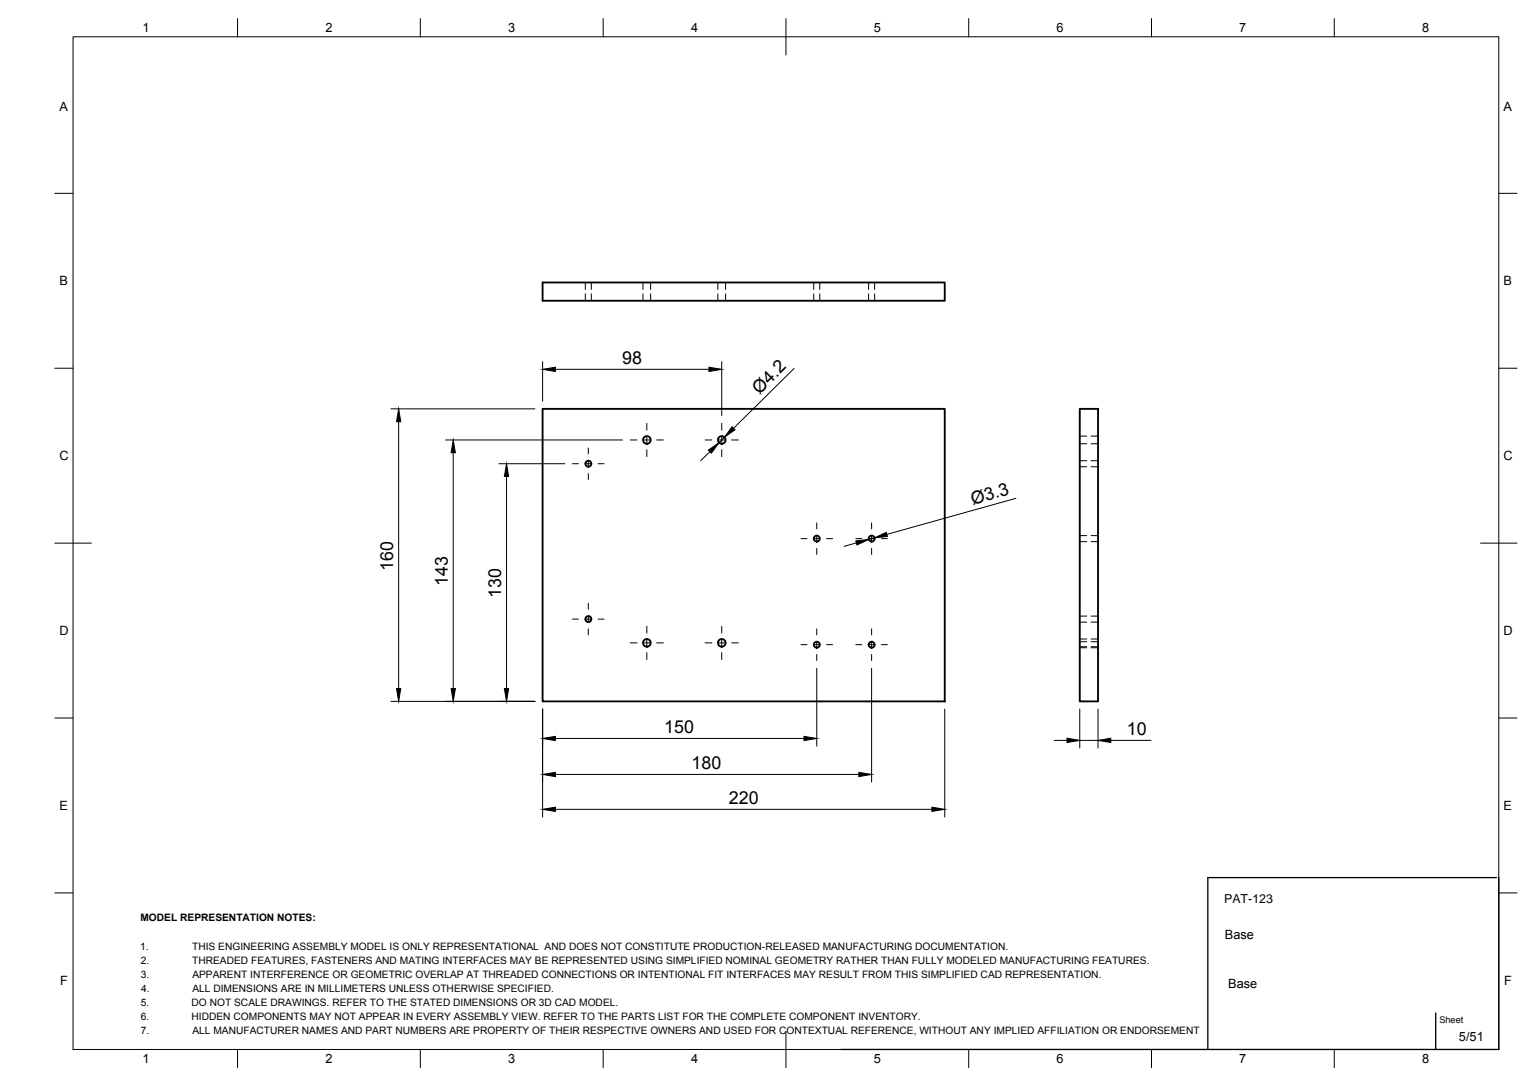
ISO-10303-21;
HEADER;
/* Generated by software containing ST-Developer
 * from STEP Tools, Inc. (www.steptools.com) 
 */

FILE_DESCRIPTION(
/* description */ ('Worm-less right-angle friction wheel drive'),
/* implementation_level */ '2;1');

FILE_NAME(
/* name */ 'Base.step',
/* time_stamp */ '2026-10-28T03:22:36-07:00',
/* author */ (''),
/* organization */ (''),
/* preprocessor_version */ 'ST-DEVELOPER v20.2',
/* originating_system */ 'Autodesk Translation Framework v15.17.0.0',
/* authorisation */ '');

FILE_SCHEMA (('AUTOMOTIVE_DESIGN { 1 0 10303 214 3 1 1 }'));
ENDSEC;

DATA;
#10=MECHANICAL_DESIGN_GEOMETRIC_PRESENTATION_REPRESENTATION('',(#611),#17046);
#517=SHAPE_REPRESENTATION_RELATIONSHIP('SRR','None',#17260,#564);
#564=ADVANCED_BREP_SHAPE_REPRESENTATION('',(#665),#16996);
#611=STYLED_ITEM('',(#17570),#665);
#665=MANIFOLD_SOLID_BREP('Body1',#8166);
#715=FACE_BOUND('',#1689,.T.);
#716=FACE_BOUND('',#1690,.T.);
#717=FACE_BOUND('',#1691,.T.);
#718=FACE_BOUND('',#1692,.T.);
#719=FACE_BOUND('',#1693,.T.);
#720=FACE_BOUND('',#1694,.T.);
#721=FACE_BOUND('',#1695,.T.);
#722=FACE_BOUND('',#1696,.T.);
#723=FACE_BOUND('',#1697,.T.);
#724=FACE_BOUND('',#1698,.T.);
#725=FACE_BOUND('',#1700,.T.);
#726=FACE_BOUND('',#1701,.T.);
#727=FACE_BOUND('',#1702,.T.);
#728=FACE_BOUND('',#1703,.T.);
#729=FACE_BOUND('',#1704,.T.);
#730=FACE_BOUND('',#1705,.T.);
#731=FACE_BOUND('',#1706,.T.);
#732=FACE_BOUND('',#1707,.T.);
#733=FACE_BOUND('',#1708,.T.);
#734=FACE_BOUND('',#1709,.T.);
#952=PLANE('',#8775);
#953=PLANE('',#8776);
#954=PLANE('',#8777);
#955=PLANE('',#8778);
#956=PLANE('',#8779);
#957=PLANE('',#8780);
#1208=FACE_OUTER_BOUND('',#1674,.T.);
#1209=FACE_OUTER_BOUND('',#1675,.T.);
#1210=FACE_OUTER_BOUND('',#1676,.T.);
#1211=FACE_OUTER_BOUND('',#1677,.T.);
#1212=FACE_OUTER_BOUND('',#1678,.T.);
#1213=FACE_OUTER_BOUND('',#1679,.T.);
#1214=FACE_OUTER_BOUND('',#1680,.T.);
#1215=FACE_OUTER_BOUND('',#1681,.T.);
#1216=FACE_OUTER_BOUND('',#1682,.T.);
#1217=FACE_OUTER_BOUND('',#1683,.T.);
#1218=FACE_OUTER_BOUND('',#1684,.T.);
#1219=FACE_OUTER_BOUND('',#1685,.T.);
#1220=FACE_OUTER_BOUND('',#1686,.T.);
#1221=FACE_OUTER_BOUND('',#1687,.T.);
#1222=FACE_OUTER_BOUND('',#1688,.T.);
#1223=FACE_OUTER_BOUND('',#1699,.T.);
#1674=EDGE_LOOP('',(#5534,#5535,#5536,#5537));
#1675=EDGE_LOOP('',(#5538,#5539,#5540,#5541));
#1676=EDGE_LOOP('',(#5542,#5543,#5544,#5545));
#1677=EDGE_LOOP('',(#5546,#5547,#5548,#5549));
#1678=EDGE_LOOP('',(#5550,#5551,#5552,#5553));
#1679=EDGE_LOOP('',(#5554,#5555,#5556,#5557));
#1680=EDGE_LOOP('',(#5558,#5559,#5560,#5561));
#1681=EDGE_LOOP('',(#5562,#5563,#5564,#5565));
#1682=EDGE_LOOP('',(#5566,#5567,#5568,#5569));
#1683=EDGE_LOOP('',(#5570,#5571,#5572,#5573));
#1684=EDGE_LOOP('',(#5574,#5575,#5576,#5577));
#1685=EDGE_LOOP('',(#5578,#5579,#5580,#5581));
#1686=EDGE_LOOP('',(#5582,#5583,#5584,#5585));
#1687=EDGE_LOOP('',(#5586,#5587,#5588,#5589));
#1688=EDGE_LOOP('',(#5590,#5591,#5592,#5593));
#1689=EDGE_LOOP('',(#5594));
#1690=EDGE_LOOP('',(#5595));
#1691=EDGE_LOOP('',(#5596));
#1692=EDGE_LOOP('',(#5597));
#1693=EDGE_LOOP('',(#5598));
#1694=EDGE_LOOP('',(#5599));
#1695=EDGE_LOOP('',(#5600));
#1696=EDGE_LOOP('',(#5601));
#1697=EDGE_LOOP('',(#5602));
#1698=EDGE_LOOP('',(#5603));
#1699=EDGE_LOOP('',(#5604,#5605,#5606,#5607));
#1700=EDGE_LOOP('',(#5608));
#1701=EDGE_LOOP('',(#5609));
#1702=EDGE_LOOP('',(#5610));
#1703=EDGE_LOOP('',(#5611));
#1704=EDGE_LOOP('',(#5612));
#1705=EDGE_LOOP('',(#5613));
#1706=EDGE_LOOP('',(#5614));
#1707=EDGE_LOOP('',(#5615));
#1708=EDGE_LOOP('',(#5616));
#1709=EDGE_LOOP('',(#5617));
#2377=LINE('',#12382,#2917);
#2378=LINE('',#12388,#2918);
#2379=LINE('',#12394,#2919);
#2380=LINE('',#12400,#2920);
#2381=LINE('',#12406,#2921);
#2382=LINE('',#12412,#2922);
#2383=LINE('',#12418,#2923);
#2384=LINE('',#12424,#2924);
#2385=LINE('',#12430,#2925);
#2386=LINE('',#12436,#2926);
#2387=LINE('',#12441,#2927);
#2388=LINE('',#12443,#2928);
#2389=LINE('',#12445,#2929);
#2390=LINE('',#12446,#2930);
#2391=LINE('',#12449,#2931);
#2392=LINE('',#12451,#2932);
#2393=LINE('',#12452,#2933);
#2394=LINE('',#12455,#2934);
#2395=LINE('',#12457,#2935);
#2396=LINE('',#12458,#2936);
#2397=LINE('',#12460,#2937);
#2398=LINE('',#12461,#2938);
#2917=VECTOR('',#9783,0.165);
#2918=VECTOR('',#9790,0.165);
#2919=VECTOR('',#9797,0.165);
#2920=VECTOR('',#9804,0.165);
#2921=VECTOR('',#9811,0.165);
#2922=VECTOR('',#9818,0.165);
#2923=VECTOR('',#9825,0.210000000000001);
#2924=VECTOR('',#9832,0.21);
#2925=VECTOR('',#9839,0.21);
#2926=VECTOR('',#9846,0.210000000000001);
#2927=VECTOR('',#9851,1.);
#2928=VECTOR('',#9852,1.);
#2929=VECTOR('',#9853,1.);
#2930=VECTOR('',#9854,1.);
#2931=VECTOR('',#9857,1.);
#2932=VECTOR('',#9858,1.);
#2933=VECTOR('',#9859,1.);
#2934=VECTOR('',#9862,1.);
#2935=VECTOR('',#9863,1.);
#2936=VECTOR('',#9864,1.);
#2937=VECTOR('',#9867,1.);
#2938=VECTOR('',#9868,1.);
#3457=CIRCLE('',#8746,0.165);
#3458=CIRCLE('',#8747,0.165);
#3459=CIRCLE('',#8749,0.165);
#3460=CIRCLE('',#8750,0.165);
#3461=CIRCLE('',#8752,0.165);
#3462=CIRCLE('',#8753,0.165);
#3463=CIRCLE('',#8755,0.165);
#3464=CIRCLE('',#8756,0.165);
#3465=CIRCLE('',#8758,0.165);
#3466=CIRCLE('',#8759,0.165);
#3467=CIRCLE('',#8761,0.165);
#3468=CIRCLE('',#8762,0.165);
#3469=CIRCLE('',#8764,0.210000000000001);
#3470=CIRCLE('',#8765,0.210000000000001);
#3471=CIRCLE('',#8767,0.21);
#3472=CIRCLE('',#8768,0.21);
#3473=CIRCLE('',#8770,0.21);
#3474=CIRCLE('',#8771,0.21);
#3475=CIRCLE('',#8773,0.210000000000001);
#3476=CIRCLE('',#8774,0.210000000000001);
#3869=VERTEX_POINT('',#12379);
#3870=VERTEX_POINT('',#12381);
#3871=VERTEX_POINT('',#12385);
#3872=VERTEX_POINT('',#12387);
#3873=VERTEX_POINT('',#12391);
#3874=VERTEX_POINT('',#12393);
#3875=VERTEX_POINT('',#12397);
#3876=VERTEX_POINT('',#12399);
#3877=VERTEX_POINT('',#12403);
#3878=VERTEX_POINT('',#12405);
#3879=VERTEX_POINT('',#12409);
#3880=VERTEX_POINT('',#12411);
#3881=VERTEX_POINT('',#12415);
#3882=VERTEX_POINT('',#12417);
#3883=VERTEX_POINT('',#12421);
#3884=VERTEX_POINT('',#12423);
#3885=VERTEX_POINT('',#12427);
#3886=VERTEX_POINT('',#12429);
#3887=VERTEX_POINT('',#12433);
#3888=VERTEX_POINT('',#12435);
#3889=VERTEX_POINT('',#12439);
#3890=VERTEX_POINT('',#12440);
#3891=VERTEX_POINT('',#12442);
#3892=VERTEX_POINT('',#12444);
#3893=VERTEX_POINT('',#12448);
#3894=VERTEX_POINT('',#12450);
#3895=VERTEX_POINT('',#12454);
#3896=VERTEX_POINT('',#12456);
#4536=EDGE_CURVE('',#3869,#3869,#3457,.T.);
#4537=EDGE_CURVE('',#3869,#3870,#2377,.T.);
#4538=EDGE_CURVE('',#3870,#3870,#3458,.T.);
#4539=EDGE_CURVE('',#3871,#3871,#3459,.T.);
#4540=EDGE_CURVE('',#3871,#3872,#2378,.T.);
#4541=EDGE_CURVE('',#3872,#3872,#3460,.T.);
#4542=EDGE_CURVE('',#3873,#3873,#3461,.T.);
#4543=EDGE_CURVE('',#3873,#3874,#2379,.T.);
#4544=EDGE_CURVE('',#3874,#3874,#3462,.T.);
#4545=EDGE_CURVE('',#3875,#3875,#3463,.T.);
#4546=EDGE_CURVE('',#3875,#3876,#2380,.T.);
#4547=EDGE_CURVE('',#3876,#3876,#3464,.T.);
#4548=EDGE_CURVE('',#3877,#3877,#3465,.T.);
#4549=EDGE_CURVE('',#3877,#3878,#2381,.T.);
#4550=EDGE_CURVE('',#3878,#3878,#3466,.T.);
#4551=EDGE_CURVE('',#3879,#3879,#3467,.T.);
#4552=EDGE_CURVE('',#3879,#3880,#2382,.T.);
#4553=EDGE_CURVE('',#3880,#3880,#3468,.T.);
#4554=EDGE_CURVE('',#3881,#3881,#3469,.T.);
#4555=EDGE_CURVE('',#3881,#3882,#2383,.T.);
#4556=EDGE_CURVE('',#3882,#3882,#3470,.T.);
#4557=EDGE_CURVE('',#3883,#3883,#3471,.T.);
#4558=EDGE_CURVE('',#3883,#3884,#2384,.T.);
#4559=EDGE_CURVE('',#3884,#3884,#3472,.T.);
#4560=EDGE_CURVE('',#3885,#3885,#3473,.T.);
#4561=EDGE_CURVE('',#3885,#3886,#2385,.T.);
#4562=EDGE_CURVE('',#3886,#3886,#3474,.T.);
#4563=EDGE_CURVE('',#3887,#3887,#3475,.T.);
#4564=EDGE_CURVE('',#3887,#3888,#2386,.T.);
#4565=EDGE_CURVE('',#3888,#3888,#3476,.T.);
#4566=EDGE_CURVE('',#3889,#3890,#2387,.T.);
#4567=EDGE_CURVE('',#3890,#3891,#2388,.T.);
#4568=EDGE_CURVE('',#3892,#3891,#2389,.T.);
#4569=EDGE_CURVE('',#3889,#3892,#2390,.T.);
#4570=EDGE_CURVE('',#3893,#3889,#2391,.T.);
#4571=EDGE_CURVE('',#3894,#3892,#2392,.T.);
#4572=EDGE_CURVE('',#3893,#3894,#2393,.T.);
#4573=EDGE_CURVE('',#3895,#3893,#2394,.T.);
#4574=EDGE_CURVE('',#3896,#3894,#2395,.T.);
#4575=EDGE_CURVE('',#3895,#3896,#2396,.T.);
#4576=EDGE_CURVE('',#3890,#3895,#2397,.T.);
#4577=EDGE_CURVE('',#3891,#3896,#2398,.T.);
#5534=ORIENTED_EDGE('',*,*,#4536,.F.);
#5535=ORIENTED_EDGE('',*,*,#4537,.T.);
#5536=ORIENTED_EDGE('',*,*,#4538,.F.);
#5537=ORIENTED_EDGE('',*,*,#4537,.F.);
#5538=ORIENTED_EDGE('',*,*,#4539,.F.);
#5539=ORIENTED_EDGE('',*,*,#4540,.T.);
#5540=ORIENTED_EDGE('',*,*,#4541,.F.);
#5541=ORIENTED_EDGE('',*,*,#4540,.F.);
#5542=ORIENTED_EDGE('',*,*,#4542,.F.);
#5543=ORIENTED_EDGE('',*,*,#4543,.T.);
#5544=ORIENTED_EDGE('',*,*,#4544,.F.);
#5545=ORIENTED_EDGE('',*,*,#4543,.F.);
#5546=ORIENTED_EDGE('',*,*,#4545,.F.);
#5547=ORIENTED_EDGE('',*,*,#4546,.T.);
#5548=ORIENTED_EDGE('',*,*,#4547,.F.);
#5549=ORIENTED_EDGE('',*,*,#4546,.F.);
#5550=ORIENTED_EDGE('',*,*,#4548,.F.);
#5551=ORIENTED_EDGE('',*,*,#4549,.T.);
#5552=ORIENTED_EDGE('',*,*,#4550,.F.);
#5553=ORIENTED_EDGE('',*,*,#4549,.F.);
#5554=ORIENTED_EDGE('',*,*,#4551,.F.);
#5555=ORIENTED_EDGE('',*,*,#4552,.T.);
#5556=ORIENTED_EDGE('',*,*,#4553,.F.);
#5557=ORIENTED_EDGE('',*,*,#4552,.F.);
#5558=ORIENTED_EDGE('',*,*,#4554,.F.);
#5559=ORIENTED_EDGE('',*,*,#4555,.T.);
#5560=ORIENTED_EDGE('',*,*,#4556,.F.);
#5561=ORIENTED_EDGE('',*,*,#4555,.F.);
#5562=ORIENTED_EDGE('',*,*,#4557,.F.);
#5563=ORIENTED_EDGE('',*,*,#4558,.T.);
#5564=ORIENTED_EDGE('',*,*,#4559,.F.);
#5565=ORIENTED_EDGE('',*,*,#4558,.F.);
#5566=ORIENTED_EDGE('',*,*,#4560,.F.);
#5567=ORIENTED_EDGE('',*,*,#4561,.T.);
#5568=ORIENTED_EDGE('',*,*,#4562,.F.);
#5569=ORIENTED_EDGE('',*,*,#4561,.F.);
#5570=ORIENTED_EDGE('',*,*,#4563,.F.);
#5571=ORIENTED_EDGE('',*,*,#4564,.T.);
#5572=ORIENTED_EDGE('',*,*,#4565,.F.);
#5573=ORIENTED_EDGE('',*,*,#4564,.F.);
#5574=ORIENTED_EDGE('',*,*,#4566,.T.);
#5575=ORIENTED_EDGE('',*,*,#4567,.T.);
#5576=ORIENTED_EDGE('',*,*,#4568,.F.);
#5577=ORIENTED_EDGE('',*,*,#4569,.F.);
#5578=ORIENTED_EDGE('',*,*,#4570,.T.);
#5579=ORIENTED_EDGE('',*,*,#4569,.T.);
#5580=ORIENTED_EDGE('',*,*,#4571,.F.);
#5581=ORIENTED_EDGE('',*,*,#4572,.F.);
#5582=ORIENTED_EDGE('',*,*,#4573,.T.);
#5583=ORIENTED_EDGE('',*,*,#4572,.T.);
#5584=ORIENTED_EDGE('',*,*,#4574,.F.);
#5585=ORIENTED_EDGE('',*,*,#4575,.F.);
#5586=ORIENTED_EDGE('',*,*,#4576,.T.);
#5587=ORIENTED_EDGE('',*,*,#4575,.T.);
#5588=ORIENTED_EDGE('',*,*,#4577,.F.);
#5589=ORIENTED_EDGE('',*,*,#4567,.F.);
#5590=ORIENTED_EDGE('',*,*,#4577,.T.);
#5591=ORIENTED_EDGE('',*,*,#4574,.T.);
#5592=ORIENTED_EDGE('',*,*,#4571,.T.);
#5593=ORIENTED_EDGE('',*,*,#4568,.T.);
#5594=ORIENTED_EDGE('',*,*,#4541,.T.);
#5595=ORIENTED_EDGE('',*,*,#4565,.T.);
#5596=ORIENTED_EDGE('',*,*,#4562,.T.);
#5597=ORIENTED_EDGE('',*,*,#4559,.T.);
#5598=ORIENTED_EDGE('',*,*,#4556,.T.);
#5599=ORIENTED_EDGE('',*,*,#4553,.T.);
#5600=ORIENTED_EDGE('',*,*,#4550,.T.);
#5601=ORIENTED_EDGE('',*,*,#4547,.T.);
#5602=ORIENTED_EDGE('',*,*,#4544,.T.);
#5603=ORIENTED_EDGE('',*,*,#4538,.T.);
#5604=ORIENTED_EDGE('',*,*,#4576,.F.);
#5605=ORIENTED_EDGE('',*,*,#4566,.F.);
#5606=ORIENTED_EDGE('',*,*,#4570,.F.);
#5607=ORIENTED_EDGE('',*,*,#4573,.F.);
#5608=ORIENTED_EDGE('',*,*,#4539,.T.);
#5609=ORIENTED_EDGE('',*,*,#4563,.T.);
#5610=ORIENTED_EDGE('',*,*,#4560,.T.);
#5611=ORIENTED_EDGE('',*,*,#4557,.T.);
#5612=ORIENTED_EDGE('',*,*,#4554,.T.);
#5613=ORIENTED_EDGE('',*,*,#4551,.T.);
#5614=ORIENTED_EDGE('',*,*,#4548,.T.);
#5615=ORIENTED_EDGE('',*,*,#4545,.T.);
#5616=ORIENTED_EDGE('',*,*,#4542,.T.);
#5617=ORIENTED_EDGE('',*,*,#4536,.T.);
#7530=CYLINDRICAL_SURFACE('',#8745,0.165);
#7531=CYLINDRICAL_SURFACE('',#8748,0.165);
#7532=CYLINDRICAL_SURFACE('',#8751,0.165);
#7533=CYLINDRICAL_SURFACE('',#8754,0.165);
#7534=CYLINDRICAL_SURFACE('',#8757,0.165);
#7535=CYLINDRICAL_SURFACE('',#8760,0.165);
#7536=CYLINDRICAL_SURFACE('',#8763,0.210000000000001);
#7537=CYLINDRICAL_SURFACE('',#8766,0.21);
#7538=CYLINDRICAL_SURFACE('',#8769,0.21);
#7539=CYLINDRICAL_SURFACE('',#8772,0.210000000000001);
#7700=ADVANCED_FACE('',(#1208),#7530,.F.);
#7701=ADVANCED_FACE('',(#1209),#7531,.F.);
#7702=ADVANCED_FACE('',(#1210),#7532,.F.);
#7703=ADVANCED_FACE('',(#1211),#7533,.F.);
#7704=ADVANCED_FACE('',(#1212),#7534,.F.);
#7705=ADVANCED_FACE('',(#1213),#7535,.F.);
#7706=ADVANCED_FACE('',(#1214),#7536,.F.);
#7707=ADVANCED_FACE('',(#1215),#7537,.F.);
#7708=ADVANCED_FACE('',(#1216),#7538,.F.);
#7709=ADVANCED_FACE('',(#1217),#7539,.F.);
#7710=ADVANCED_FACE('',(#1218),#952,.T.);
#7711=ADVANCED_FACE('',(#1219),#953,.T.);
#7712=ADVANCED_FACE('',(#1220),#954,.T.);
#7713=ADVANCED_FACE('',(#1221),#955,.T.);
#7714=ADVANCED_FACE('',(#1222,#715,#716,#717,#718,#719,#720,#721,#722,#723,
#724),#956,.T.);
#7715=ADVANCED_FACE('',(#1223,#725,#726,#727,#728,#729,#730,#731,#732,#733,
#734),#957,.F.);
#8166=CLOSED_SHELL('',(#7700,#7701,#7702,#7703,#7704,#7705,#7706,#7707,
#7708,#7709,#7710,#7711,#7712,#7713,#7714,#7715));
#8744=AXIS2_PLACEMENT_3D('',#12377,#9777,#9778);
#8745=AXIS2_PLACEMENT_3D('',#12378,#9779,#9780);
#8746=AXIS2_PLACEMENT_3D('',#12380,#9781,#9782);
#8747=AXIS2_PLACEMENT_3D('',#12383,#9784,#9785);
#8748=AXIS2_PLACEMENT_3D('',#12384,#9786,#9787);
#8749=AXIS2_PLACEMENT_3D('',#12386,#9788,#9789);
#8750=AXIS2_PLACEMENT_3D('',#12389,#9791,#9792);
#8751=AXIS2_PLACEMENT_3D('',#12390,#9793,#9794);
#8752=AXIS2_PLACEMENT_3D('',#12392,#9795,#9796);
#8753=AXIS2_PLACEMENT_3D('',#12395,#9798,#9799);
#8754=AXIS2_PLACEMENT_3D('',#12396,#9800,#9801);
#8755=AXIS2_PLACEMENT_3D('',#12398,#9802,#9803);
#8756=AXIS2_PLACEMENT_3D('',#12401,#9805,#9806);
#8757=AXIS2_PLACEMENT_3D('',#12402,#9807,#9808);
#8758=AXIS2_PLACEMENT_3D('',#12404,#9809,#9810);
#8759=AXIS2_PLACEMENT_3D('',#12407,#9812,#9813);
#8760=AXIS2_PLACEMENT_3D('',#12408,#9814,#9815);
#8761=AXIS2_PLACEMENT_3D('',#12410,#9816,#9817);
#8762=AXIS2_PLACEMENT_3D('',#12413,#9819,#9820);
#8763=AXIS2_PLACEMENT_3D('',#12414,#9821,#9822);
#8764=AXIS2_PLACEMENT_3D('',#12416,#9823,#9824);
#8765=AXIS2_PLACEMENT_3D('',#12419,#9826,#9827);
#8766=AXIS2_PLACEMENT_3D('',#12420,#9828,#9829);
#8767=AXIS2_PLACEMENT_3D('',#12422,#9830,#9831);
#8768=AXIS2_PLACEMENT_3D('',#12425,#9833,#9834);
#8769=AXIS2_PLACEMENT_3D('',#12426,#9835,#9836);
#8770=AXIS2_PLACEMENT_3D('',#12428,#9837,#9838);
#8771=AXIS2_PLACEMENT_3D('',#12431,#9840,#9841);
#8772=AXIS2_PLACEMENT_3D('',#12432,#9842,#9843);
#8773=AXIS2_PLACEMENT_3D('',#12434,#9844,#9845);
#8774=AXIS2_PLACEMENT_3D('',#12437,#9847,#9848);
#8775=AXIS2_PLACEMENT_3D('',#12438,#9849,#9850);
#8776=AXIS2_PLACEMENT_3D('',#12447,#9855,#9856);
#8777=AXIS2_PLACEMENT_3D('',#12453,#9860,#9861);
#8778=AXIS2_PLACEMENT_3D('',#12459,#9865,#9866);
#8779=AXIS2_PLACEMENT_3D('',#12462,#9869,#9870);
#8780=AXIS2_PLACEMENT_3D('',#12463,#9871,#9872);
#9777=DIRECTION('axis',(0.,0.,1.));
#9778=DIRECTION('refdir',(1.,0.,0.));
#9779=DIRECTION('center_axis',(0.,0.,1.));
#9780=DIRECTION('ref_axis',(1.,0.,0.));
#9781=DIRECTION('center_axis',(0.,0.,1.));
#9782=DIRECTION('ref_axis',(1.,0.,0.));
#9783=DIRECTION('',(0.,0.,1.));
#9784=DIRECTION('center_axis',(0.,0.,-1.));
#9785=DIRECTION('ref_axis',(1.,0.,0.));
#9786=DIRECTION('center_axis',(0.,0.,1.));
#9787=DIRECTION('ref_axis',(1.,0.,0.));
#9788=DIRECTION('center_axis',(0.,0.,1.));
#9789=DIRECTION('ref_axis',(1.,0.,0.));
#9790=DIRECTION('',(0.,0.,1.));
#9791=DIRECTION('center_axis',(0.,0.,-1.));
#9792=DIRECTION('ref_axis',(1.,0.,0.));
#9793=DIRECTION('center_axis',(0.,0.,1.));
#9794=DIRECTION('ref_axis',(1.,0.,0.));
#9795=DIRECTION('center_axis',(0.,0.,1.));
#9796=DIRECTION('ref_axis',(1.,0.,0.));
#9797=DIRECTION('',(0.,0.,1.));
#9798=DIRECTION('center_axis',(0.,0.,-1.));
#9799=DIRECTION('ref_axis',(1.,0.,0.));
#9800=DIRECTION('center_axis',(0.,0.,1.));
#9801=DIRECTION('ref_axis',(1.,0.,0.));
#9802=DIRECTION('center_axis',(0.,0.,1.));
#9803=DIRECTION('ref_axis',(1.,0.,0.));
#9804=DIRECTION('',(0.,0.,1.));
#9805=DIRECTION('center_axis',(0.,0.,-1.));
#9806=DIRECTION('ref_axis',(1.,0.,0.));
#9807=DIRECTION('center_axis',(0.,0.,1.));
#9808=DIRECTION('ref_axis',(1.,0.,0.));
#9809=DIRECTION('center_axis',(0.,0.,1.));
#9810=DIRECTION('ref_axis',(1.,0.,0.));
#9811=DIRECTION('',(0.,0.,1.));
#9812=DIRECTION('center_axis',(0.,0.,-1.));
#9813=DIRECTION('ref_axis',(1.,0.,0.));
#9814=DIRECTION('center_axis',(0.,0.,1.));
#9815=DIRECTION('ref_axis',(1.,0.,0.));
#9816=DIRECTION('center_axis',(0.,0.,1.));
#9817=DIRECTION('ref_axis',(1.,0.,0.));
#9818=DIRECTION('',(0.,0.,1.));
#9819=DIRECTION('center_axis',(0.,0.,-1.));
#9820=DIRECTION('ref_axis',(1.,0.,0.));
#9821=DIRECTION('center_axis',(0.,0.,1.));
#9822=DIRECTION('ref_axis',(1.,0.,0.));
#9823=DIRECTION('center_axis',(0.,0.,1.));
#9824=DIRECTION('ref_axis',(1.,0.,0.));
#9825=DIRECTION('',(0.,0.,1.));
#9826=DIRECTION('center_axis',(0.,0.,-1.));
#9827=DIRECTION('ref_axis',(1.,0.,0.));
#9828=DIRECTION('center_axis',(0.,0.,1.));
#9829=DIRECTION('ref_axis',(1.,0.,0.));
#9830=DIRECTION('center_axis',(0.,0.,1.));
#9831=DIRECTION('ref_axis',(1.,0.,0.));
#9832=DIRECTION('',(0.,0.,1.));
#9833=DIRECTION('center_axis',(0.,0.,-1.));
#9834=DIRECTION('ref_axis',(1.,0.,0.));
#9835=DIRECTION('center_axis',(0.,0.,1.));
#9836=DIRECTION('ref_axis',(1.,0.,0.));
#9837=DIRECTION('center_axis',(0.,0.,1.));
#9838=DIRECTION('ref_axis',(1.,0.,0.));
#9839=DIRECTION('',(0.,0.,1.));
#9840=DIRECTION('center_axis',(0.,0.,-1.));
#9841=DIRECTION('ref_axis',(1.,0.,0.));
#9842=DIRECTION('center_axis',(0.,0.,1.));
#9843=DIRECTION('ref_axis',(1.,0.,0.));
#9844=DIRECTION('center_axis',(0.,0.,1.));
#9845=DIRECTION('ref_axis',(1.,0.,0.));
#9846=DIRECTION('',(0.,0.,1.));
#9847=DIRECTION('center_axis',(0.,0.,-1.));
#9848=DIRECTION('ref_axis',(1.,0.,0.));
#9849=DIRECTION('center_axis',(0.,1.,0.));
#9850=DIRECTION('ref_axis',(-1.,0.,0.));
#9851=DIRECTION('',(-1.,0.,0.));
#9852=DIRECTION('',(0.,0.,1.));
#9853=DIRECTION('',(-1.,0.,0.));
#9854=DIRECTION('',(0.,0.,1.));
#9855=DIRECTION('center_axis',(1.,0.,0.));
#9856=DIRECTION('ref_axis',(0.,1.,0.));
#9857=DIRECTION('',(0.,1.,0.));
#9858=DIRECTION('',(0.,1.,0.));
#9859=DIRECTION('',(0.,0.,1.));
#9860=DIRECTION('center_axis',(0.,-1.,0.));
#9861=DIRECTION('ref_axis',(1.,0.,0.));
#9862=DIRECTION('',(1.,0.,0.));
#9863=DIRECTION('',(1.,0.,0.));
#9864=DIRECTION('',(0.,0.,1.));
#9865=DIRECTION('center_axis',(-1.,0.,0.));
#9866=DIRECTION('ref_axis',(0.,-1.,0.));
#9867=DIRECTION('',(0.,-1.,0.));
#9868=DIRECTION('',(0.,-1.,0.));
#9869=DIRECTION('center_axis',(0.,0.,1.));
#9870=DIRECTION('ref_axis',(1.,0.,0.));
#9871=DIRECTION('center_axis',(0.,0.,1.));
#9872=DIRECTION('ref_axis',(1.,0.,0.));
#12377=CARTESIAN_POINT('',(0.,0.,0.));
#12378=CARTESIAN_POINT('Origin',(7.,8.5,-0.1));
#12379=CARTESIAN_POINT('',(6.835,8.5,0.));
#12380=CARTESIAN_POINT('Origin',(7.,8.5,0.));
#12381=CARTESIAN_POINT('',(6.835,8.5,1.));
#12382=CARTESIAN_POINT('',(6.835,8.5,-0.1));
#12383=CARTESIAN_POINT('Origin',(7.,8.5,1.));
#12384=CARTESIAN_POINT('Origin',(-1.5,8.5,-0.1));
#12385=CARTESIAN_POINT('',(-1.665,8.5,0.));
#12386=CARTESIAN_POINT('Origin',(-1.5,8.5,0.));
#12387=CARTESIAN_POINT('',(-1.665,8.5,1.));
#12388=CARTESIAN_POINT('',(-1.665,8.5,-0.1));
#12389=CARTESIAN_POINT('Origin',(-1.5,8.5,1.));
#12390=CARTESIAN_POINT('Origin',(-2.9,-4.,-0.1));
#12391=CARTESIAN_POINT('',(-3.065,-4.,0.));
#12392=CARTESIAN_POINT('Origin',(-2.9,-4.,0.));
#12393=CARTESIAN_POINT('',(-3.065,-4.,1.));
#12394=CARTESIAN_POINT('',(-3.065,-4.,-0.1));
#12395=CARTESIAN_POINT('Origin',(-2.9,-4.,1.));
#12396=CARTESIAN_POINT('Origin',(2.9,-4.,-0.1));
#12397=CARTESIAN_POINT('',(2.735,-4.,0.));
#12398=CARTESIAN_POINT('Origin',(2.9,-4.,0.));
#12399=CARTESIAN_POINT('',(2.735,-4.,1.));
#12400=CARTESIAN_POINT('',(2.735,-4.,-0.1));
#12401=CARTESIAN_POINT('Origin',(2.9,-4.,1.));
#12402=CARTESIAN_POINT('Origin',(-2.9,-7.,-0.1));
#12403=CARTESIAN_POINT('',(-3.065,-7.,0.));
#12404=CARTESIAN_POINT('Origin',(-2.9,-7.,0.));
#12405=CARTESIAN_POINT('',(-3.065,-7.,1.));
#12406=CARTESIAN_POINT('',(-3.065,-7.,-0.1));
#12407=CARTESIAN_POINT('Origin',(-2.9,-7.,1.));
#12408=CARTESIAN_POINT('Origin',(2.9,-7.,-0.1));
#12409=CARTESIAN_POINT('',(2.735,-7.,0.));
#12410=CARTESIAN_POINT('Origin',(2.9,-7.,0.));
#12411=CARTESIAN_POINT('',(2.735,-7.,1.));
#12412=CARTESIAN_POINT('',(2.735,-7.,-0.1));
#12413=CARTESIAN_POINT('Origin',(2.9,-7.,1.));
#12414=CARTESIAN_POINT('Origin',(8.3,1.2,-0.1));
#12415=CARTESIAN_POINT('',(8.09,1.2,0.));
#12416=CARTESIAN_POINT('Origin',(8.3,1.2,0.));
#12417=CARTESIAN_POINT('',(8.09,1.2,1.));
#12418=CARTESIAN_POINT('',(8.09,1.2,-0.1));
#12419=CARTESIAN_POINT('Origin',(8.3,1.2,1.));
#12420=CARTESIAN_POINT('Origin',(-2.8,5.3,-0.1));
#12421=CARTESIAN_POINT('',(-3.01,5.3,0.));
#12422=CARTESIAN_POINT('Origin',(-2.8,5.3,0.));
#12423=CARTESIAN_POINT('',(-3.01,5.3,1.));
#12424=CARTESIAN_POINT('',(-3.01,5.3,-0.1));
#12425=CARTESIAN_POINT('Origin',(-2.8,5.3,1.));
#12426=CARTESIAN_POINT('Origin',(-2.8,1.2,-0.1));
#12427=CARTESIAN_POINT('',(-3.01,1.2,0.));
#12428=CARTESIAN_POINT('Origin',(-2.8,1.2,0.));
#12429=CARTESIAN_POINT('',(-3.01,1.2,1.));
#12430=CARTESIAN_POINT('',(-3.01,1.2,-0.1));
#12431=CARTESIAN_POINT('Origin',(-2.8,1.2,1.));
#12432=CARTESIAN_POINT('Origin',(8.3,5.3,-0.1));
#12433=CARTESIAN_POINT('',(8.09,5.3,0.));
#12434=CARTESIAN_POINT('Origin',(8.3,5.3,0.));
#12435=CARTESIAN_POINT('',(8.09,5.3,1.));
#12436=CARTESIAN_POINT('',(8.09,5.3,-0.1));
#12437=CARTESIAN_POINT('Origin',(8.3,5.3,1.));
#12438=CARTESIAN_POINT('Origin',(10.,11.,0.));
#12439=CARTESIAN_POINT('',(10.,11.,0.));
#12440=CARTESIAN_POINT('',(-6.,11.,0.));
#12441=CARTESIAN_POINT('',(10.,11.,0.));
#12442=CARTESIAN_POINT('',(-6.,11.,1.));
#12443=CARTESIAN_POINT('',(-6.,11.,0.));
#12444=CARTESIAN_POINT('',(10.,11.,1.));
#12445=CARTESIAN_POINT('',(10.,11.,1.));
#12446=CARTESIAN_POINT('',(10.,11.,0.));
#12447=CARTESIAN_POINT('Origin',(10.,-11.,0.));
#12448=CARTESIAN_POINT('',(10.,-11.,0.));
#12449=CARTESIAN_POINT('',(10.,-11.,0.));
#12450=CARTESIAN_POINT('',(10.,-11.,1.));
#12451=CARTESIAN_POINT('',(10.,-11.,1.));
#12452=CARTESIAN_POINT('',(10.,-11.,0.));
#12453=CARTESIAN_POINT('Origin',(-6.,-11.,0.));
#12454=CARTESIAN_POINT('',(-6.,-11.,0.));
#12455=CARTESIAN_POINT('',(-6.,-11.,0.));
#12456=CARTESIAN_POINT('',(-6.,-11.,1.));
#12457=CARTESIAN_POINT('',(-6.,-11.,1.));
#12458=CARTESIAN_POINT('',(-6.,-11.,0.));
#12459=CARTESIAN_POINT('Origin',(-6.,11.,0.));
#12460=CARTESIAN_POINT('',(-6.,11.,0.));
#12461=CARTESIAN_POINT('',(-6.,11.,1.));
#12462=CARTESIAN_POINT('Origin',(2.,0.,1.));
#12463=CARTESIAN_POINT('Origin',(2.,0.,0.));
#16943=UNCERTAINTY_MEASURE_WITH_UNIT(LENGTH_MEASURE(0.001),#17047,
'DISTANCE_ACCURACY_VALUE',
'Maximum model space distance between geometric entities at asserted c
onnectivities');
#16993=UNCERTAINTY_MEASURE_WITH_UNIT(LENGTH_MEASURE(0.001),#17047,
'DISTANCE_ACCURACY_VALUE',
'Maximum model space distance between geometric entities at asserted c
onnectivities');
#16996=(
GEOMETRIC_REPRESENTATION_CONTEXT(3)
GLOBAL_UNCERTAINTY_ASSIGNED_CONTEXT((#16943))
GLOBAL_UNIT_ASSIGNED_CONTEXT((#17047,#17049,#17050))
REPRESENTATION_CONTEXT('','3D')
);
#17046=(
GEOMETRIC_REPRESENTATION_CONTEXT(3)
GLOBAL_UNCERTAINTY_ASSIGNED_CONTEXT((#16993))
GLOBAL_UNIT_ASSIGNED_CONTEXT((#17047,#17049,#17050))
REPRESENTATION_CONTEXT('','3D')
);
#17047=(
LENGTH_UNIT()
NAMED_UNIT(*)
SI_UNIT(.CENTI.,.METRE.)
);
#17049=(
NAMED_UNIT(*)
PLANE_ANGLE_UNIT()
SI_UNIT($,.RADIAN.)
);
#17050=(
NAMED_UNIT(*)
SI_UNIT($,.STERADIAN.)
SOLID_ANGLE_UNIT()
);
#17053=SHAPE_DEFINITION_REPRESENTATION(#17105,#17260);
#17105=PRODUCT_DEFINITION_SHAPE('',$,#17313);
#17260=SHAPE_REPRESENTATION('',(#8744),#16996);
#17310=PRODUCT_DEFINITION_CONTEXT('part definition',#17468,'design');
#17313=PRODUCT_DEFINITION('Base','Base',#17365,#17310);
#17365=PRODUCT_DEFINITION_FORMATION('',$,#17472);
#17468=APPLICATION_CONTEXT(
'Core Data for Automotive Mechanical Design Process');
#17469=PRODUCT_CONTEXT('part definition',#17468,'mechanical');
#17472=PRODUCT('Base','Base','Base',(#17469));
#17564=COLOUR_RGB('Dark Blue',0.08,0.2,0.34);
#17565=FILL_AREA_STYLE_COLOUR('',#17564);
#17566=FILL_AREA_STYLE('',(#17565));
#17567=SURFACE_STYLE_FILL_AREA(#17566);
#17568=SURFACE_SIDE_STYLE('',(#17567));
#17569=SURFACE_STYLE_USAGE(.BOTH.,#17568);
#17570=PRESENTATION_STYLE_ASSIGNMENT((#17569));
ENDSEC;
END-ISO-10303-21;
